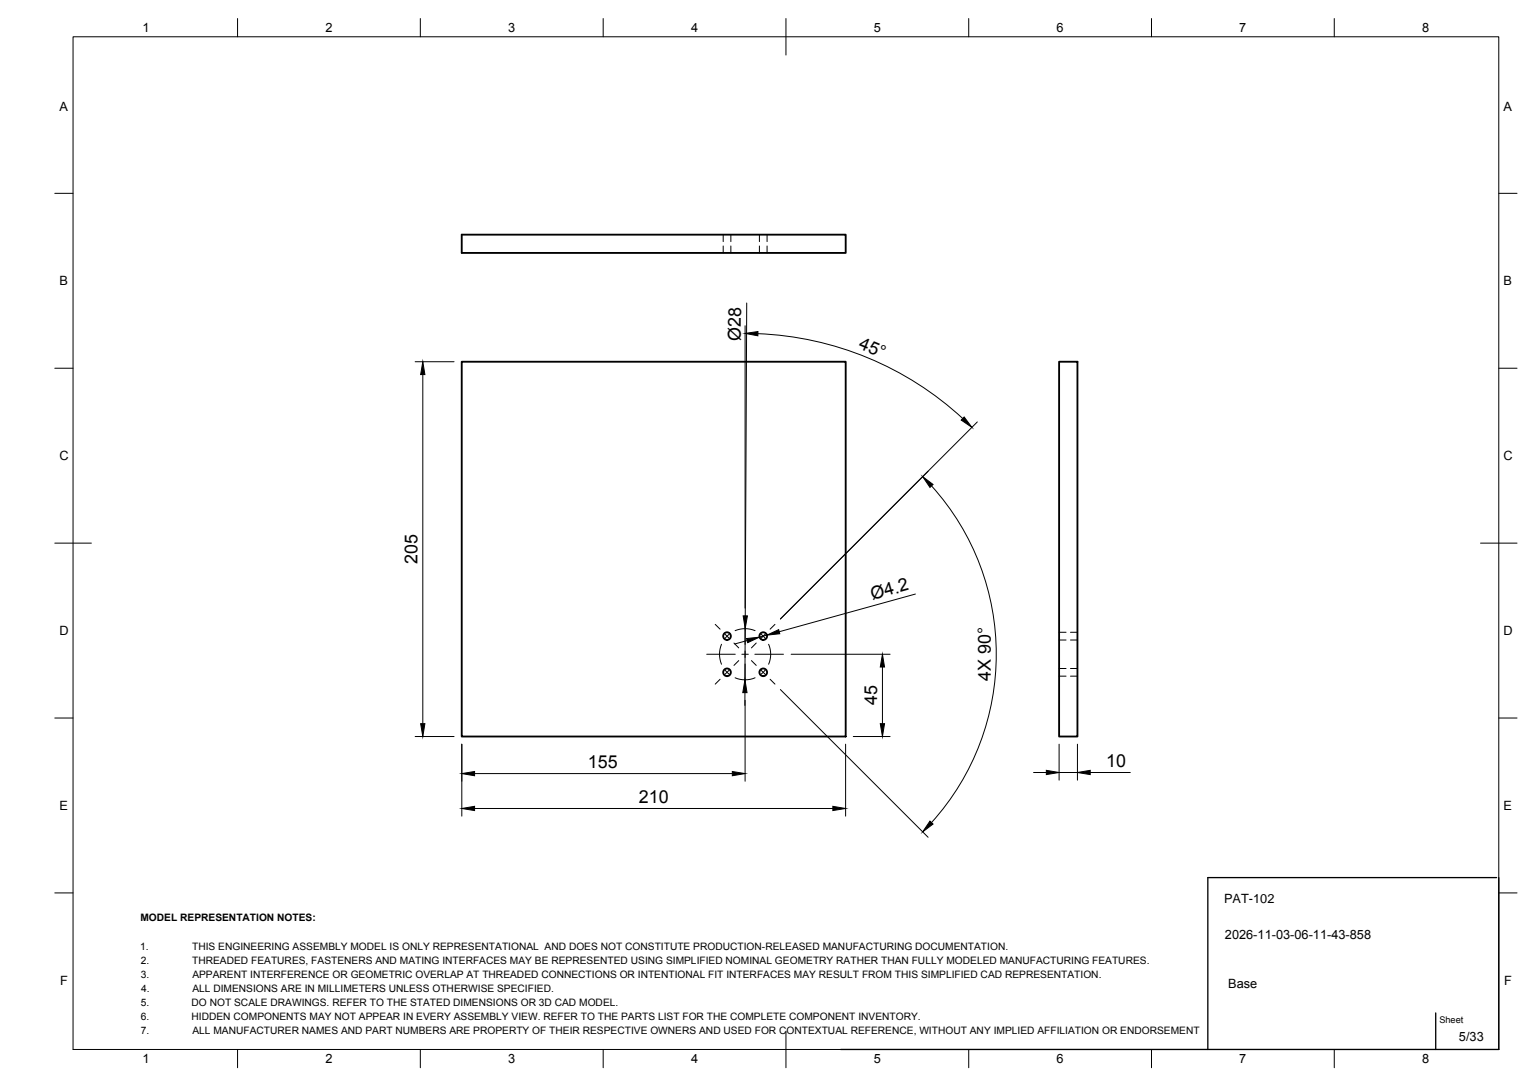
ISO-10303-21;
HEADER;
/* Generated by software containing ST-Developer
 * from STEP Tools, Inc. (www.steptools.com) 
 */

FILE_DESCRIPTION(
/* description */ ('Swing-away clamp arm'),
/* implementation_level */ '2;1');

FILE_NAME(
/* name */ 'Base.step',
/* time_stamp */ '2026-10-28T03:26:03-07:00',
/* author */ (''),
/* organization */ (''),
/* preprocessor_version */ 'ST-DEVELOPER v20.2',
/* originating_system */ 'Autodesk Translation Framework v15.17.0.0',
/* authorisation */ '');

FILE_SCHEMA (('AUTOMOTIVE_DESIGN { 1 0 10303 214 3 1 1 }'));
ENDSEC;

DATA;
#10=MECHANICAL_DESIGN_GEOMETRIC_PRESENTATION_REPRESENTATION('',(#293),#10627);
#241=SHAPE_REPRESENTATION_RELATIONSHIP('SRR','None',#10739,#267);
#267=ADVANCED_BREP_SHAPE_REPRESENTATION('',(#327),#10598);
#293=STYLED_ITEM('',(#10944),#327);
#327=MANIFOLD_SOLID_BREP('Body1',#4899);
#358=FACE_BOUND('',#953,.T.);
#359=FACE_BOUND('',#954,.T.);
#360=FACE_BOUND('',#955,.T.);
#361=FACE_BOUND('',#956,.T.);
#362=FACE_BOUND('',#958,.T.);
#363=FACE_BOUND('',#959,.T.);
#364=FACE_BOUND('',#960,.T.);
#365=FACE_BOUND('',#961,.T.);
#458=PLANE('',#5238);
#459=PLANE('',#5239);
#460=PLANE('',#5240);
#461=PLANE('',#5241);
#462=PLANE('',#5242);
#463=PLANE('',#5243);
#637=FACE_OUTER_BOUND('',#944,.T.);
#638=FACE_OUTER_BOUND('',#945,.T.);
#639=FACE_OUTER_BOUND('',#946,.T.);
#640=FACE_OUTER_BOUND('',#947,.T.);
#641=FACE_OUTER_BOUND('',#948,.T.);
#642=FACE_OUTER_BOUND('',#949,.T.);
#643=FACE_OUTER_BOUND('',#950,.T.);
#644=FACE_OUTER_BOUND('',#951,.T.);
#645=FACE_OUTER_BOUND('',#952,.T.);
#646=FACE_OUTER_BOUND('',#957,.T.);
#944=EDGE_LOOP('',(#3281,#3282,#3283,#3284));
#945=EDGE_LOOP('',(#3285,#3286,#3287,#3288));
#946=EDGE_LOOP('',(#3289,#3290,#3291,#3292));
#947=EDGE_LOOP('',(#3293,#3294,#3295,#3296));
#948=EDGE_LOOP('',(#3297,#3298,#3299,#3300));
#949=EDGE_LOOP('',(#3301,#3302,#3303,#3304));
#950=EDGE_LOOP('',(#3305,#3306,#3307,#3308));
#951=EDGE_LOOP('',(#3309,#3310,#3311,#3312));
#952=EDGE_LOOP('',(#3313,#3314,#3315,#3316));
#953=EDGE_LOOP('',(#3317));
#954=EDGE_LOOP('',(#3318));
#955=EDGE_LOOP('',(#3319));
#956=EDGE_LOOP('',(#3320));
#957=EDGE_LOOP('',(#3321,#3322,#3323,#3324));
#958=EDGE_LOOP('',(#3325));
#959=EDGE_LOOP('',(#3326));
#960=EDGE_LOOP('',(#3327));
#961=EDGE_LOOP('',(#3328));
#1351=LINE('',#7493,#1673);
#1352=LINE('',#7499,#1674);
#1353=LINE('',#7505,#1675);
#1354=LINE('',#7511,#1676);
#1355=LINE('',#7516,#1677);
#1356=LINE('',#7518,#1678);
#1357=LINE('',#7520,#1679);
#1358=LINE('',#7521,#1680);
#1359=LINE('',#7524,#1681);
#1360=LINE('',#7526,#1682);
#1361=LINE('',#7527,#1683);
#1362=LINE('',#7530,#1684);
#1363=LINE('',#7532,#1685);
#1364=LINE('',#7533,#1686);
#1365=LINE('',#7535,#1687);
#1366=LINE('',#7536,#1688);
#1673=VECTOR('',#5880,0.21);
#1674=VECTOR('',#5887,0.21);
#1675=VECTOR('',#5894,0.21);
#1676=VECTOR('',#5901,0.21);
#1677=VECTOR('',#5906,1.);
#1678=VECTOR('',#5907,1.);
#1679=VECTOR('',#5908,1.);
#1680=VECTOR('',#5909,1.);
#1681=VECTOR('',#5912,1.);
#1682=VECTOR('',#5913,1.);
#1683=VECTOR('',#5914,1.);
#1684=VECTOR('',#5917,1.);
#1685=VECTOR('',#5918,1.);
#1686=VECTOR('',#5919,1.);
#1687=VECTOR('',#5922,1.);
#1688=VECTOR('',#5923,1.);
#1995=CIRCLE('',#5227,0.21);
#1996=CIRCLE('',#5228,0.21);
#1997=CIRCLE('',#5230,0.21);
#1998=CIRCLE('',#5231,0.21);
#1999=CIRCLE('',#5233,0.21);
#2000=CIRCLE('',#5234,0.21);
#2001=CIRCLE('',#5236,0.21);
#2002=CIRCLE('',#5237,0.21);
#2262=VERTEX_POINT('',#7490);
#2263=VERTEX_POINT('',#7492);
#2264=VERTEX_POINT('',#7496);
#2265=VERTEX_POINT('',#7498);
#2266=VERTEX_POINT('',#7502);
#2267=VERTEX_POINT('',#7504);
#2268=VERTEX_POINT('',#7508);
#2269=VERTEX_POINT('',#7510);
#2270=VERTEX_POINT('',#7514);
#2271=VERTEX_POINT('',#7515);
#2272=VERTEX_POINT('',#7517);
#2273=VERTEX_POINT('',#7519);
#2274=VERTEX_POINT('',#7523);
#2275=VERTEX_POINT('',#7525);
#2276=VERTEX_POINT('',#7529);
#2277=VERTEX_POINT('',#7531);
#2673=EDGE_CURVE('',#2262,#2262,#1995,.T.);
#2674=EDGE_CURVE('',#2262,#2263,#1351,.T.);
#2675=EDGE_CURVE('',#2263,#2263,#1996,.T.);
#2676=EDGE_CURVE('',#2264,#2264,#1997,.T.);
#2677=EDGE_CURVE('',#2264,#2265,#1352,.T.);
#2678=EDGE_CURVE('',#2265,#2265,#1998,.T.);
#2679=EDGE_CURVE('',#2266,#2266,#1999,.T.);
#2680=EDGE_CURVE('',#2266,#2267,#1353,.T.);
#2681=EDGE_CURVE('',#2267,#2267,#2000,.T.);
#2682=EDGE_CURVE('',#2268,#2268,#2001,.T.);
#2683=EDGE_CURVE('',#2268,#2269,#1354,.T.);
#2684=EDGE_CURVE('',#2269,#2269,#2002,.T.);
#2685=EDGE_CURVE('',#2270,#2271,#1355,.T.);
#2686=EDGE_CURVE('',#2271,#2272,#1356,.T.);
#2687=EDGE_CURVE('',#2273,#2272,#1357,.T.);
#2688=EDGE_CURVE('',#2270,#2273,#1358,.T.);
#2689=EDGE_CURVE('',#2274,#2270,#1359,.T.);
#2690=EDGE_CURVE('',#2275,#2273,#1360,.T.);
#2691=EDGE_CURVE('',#2274,#2275,#1361,.T.);
#2692=EDGE_CURVE('',#2276,#2274,#1362,.T.);
#2693=EDGE_CURVE('',#2277,#2275,#1363,.T.);
#2694=EDGE_CURVE('',#2276,#2277,#1364,.T.);
#2695=EDGE_CURVE('',#2271,#2276,#1365,.T.);
#2696=EDGE_CURVE('',#2272,#2277,#1366,.T.);
#3281=ORIENTED_EDGE('',*,*,#2673,.F.);
#3282=ORIENTED_EDGE('',*,*,#2674,.T.);
#3283=ORIENTED_EDGE('',*,*,#2675,.F.);
#3284=ORIENTED_EDGE('',*,*,#2674,.F.);
#3285=ORIENTED_EDGE('',*,*,#2676,.F.);
#3286=ORIENTED_EDGE('',*,*,#2677,.T.);
#3287=ORIENTED_EDGE('',*,*,#2678,.F.);
#3288=ORIENTED_EDGE('',*,*,#2677,.F.);
#3289=ORIENTED_EDGE('',*,*,#2679,.F.);
#3290=ORIENTED_EDGE('',*,*,#2680,.T.);
#3291=ORIENTED_EDGE('',*,*,#2681,.F.);
#3292=ORIENTED_EDGE('',*,*,#2680,.F.);
#3293=ORIENTED_EDGE('',*,*,#2682,.F.);
#3294=ORIENTED_EDGE('',*,*,#2683,.T.);
#3295=ORIENTED_EDGE('',*,*,#2684,.F.);
#3296=ORIENTED_EDGE('',*,*,#2683,.F.);
#3297=ORIENTED_EDGE('',*,*,#2685,.T.);
#3298=ORIENTED_EDGE('',*,*,#2686,.T.);
#3299=ORIENTED_EDGE('',*,*,#2687,.F.);
#3300=ORIENTED_EDGE('',*,*,#2688,.F.);
#3301=ORIENTED_EDGE('',*,*,#2689,.T.);
#3302=ORIENTED_EDGE('',*,*,#2688,.T.);
#3303=ORIENTED_EDGE('',*,*,#2690,.F.);
#3304=ORIENTED_EDGE('',*,*,#2691,.F.);
#3305=ORIENTED_EDGE('',*,*,#2692,.T.);
#3306=ORIENTED_EDGE('',*,*,#2691,.T.);
#3307=ORIENTED_EDGE('',*,*,#2693,.F.);
#3308=ORIENTED_EDGE('',*,*,#2694,.F.);
#3309=ORIENTED_EDGE('',*,*,#2695,.T.);
#3310=ORIENTED_EDGE('',*,*,#2694,.T.);
#3311=ORIENTED_EDGE('',*,*,#2696,.F.);
#3312=ORIENTED_EDGE('',*,*,#2686,.F.);
#3313=ORIENTED_EDGE('',*,*,#2696,.T.);
#3314=ORIENTED_EDGE('',*,*,#2693,.T.);
#3315=ORIENTED_EDGE('',*,*,#2690,.T.);
#3316=ORIENTED_EDGE('',*,*,#2687,.T.);
#3317=ORIENTED_EDGE('',*,*,#2675,.T.);
#3318=ORIENTED_EDGE('',*,*,#2678,.T.);
#3319=ORIENTED_EDGE('',*,*,#2681,.T.);
#3320=ORIENTED_EDGE('',*,*,#2684,.T.);
#3321=ORIENTED_EDGE('',*,*,#2695,.F.);
#3322=ORIENTED_EDGE('',*,*,#2685,.F.);
#3323=ORIENTED_EDGE('',*,*,#2689,.F.);
#3324=ORIENTED_EDGE('',*,*,#2692,.F.);
#3325=ORIENTED_EDGE('',*,*,#2673,.T.);
#3326=ORIENTED_EDGE('',*,*,#2676,.T.);
#3327=ORIENTED_EDGE('',*,*,#2679,.T.);
#3328=ORIENTED_EDGE('',*,*,#2682,.T.);
#4497=CYLINDRICAL_SURFACE('',#5226,0.21);
#4498=CYLINDRICAL_SURFACE('',#5229,0.21);
#4499=CYLINDRICAL_SURFACE('',#5232,0.21);
#4500=CYLINDRICAL_SURFACE('',#5235,0.21);
#4592=ADVANCED_FACE('',(#637),#4497,.F.);
#4593=ADVANCED_FACE('',(#638),#4498,.F.);
#4594=ADVANCED_FACE('',(#639),#4499,.F.);
#4595=ADVANCED_FACE('',(#640),#4500,.F.);
#4596=ADVANCED_FACE('',(#641),#458,.T.);
#4597=ADVANCED_FACE('',(#642),#459,.T.);
#4598=ADVANCED_FACE('',(#643),#460,.T.);
#4599=ADVANCED_FACE('',(#644),#461,.T.);
#4600=ADVANCED_FACE('',(#645,#358,#359,#360,#361),#462,.T.);
#4601=ADVANCED_FACE('',(#646,#362,#363,#364,#365),#463,.F.);
#4899=CLOSED_SHELL('',(#4592,#4593,#4594,#4595,#4596,#4597,#4598,#4599,
#4600,#4601));
#5225=AXIS2_PLACEMENT_3D('',#7488,#5874,#5875);
#5226=AXIS2_PLACEMENT_3D('',#7489,#5876,#5877);
#5227=AXIS2_PLACEMENT_3D('',#7491,#5878,#5879);
#5228=AXIS2_PLACEMENT_3D('',#7494,#5881,#5882);
#5229=AXIS2_PLACEMENT_3D('',#7495,#5883,#5884);
#5230=AXIS2_PLACEMENT_3D('',#7497,#5885,#5886);
#5231=AXIS2_PLACEMENT_3D('',#7500,#5888,#5889);
#5232=AXIS2_PLACEMENT_3D('',#7501,#5890,#5891);
#5233=AXIS2_PLACEMENT_3D('',#7503,#5892,#5893);
#5234=AXIS2_PLACEMENT_3D('',#7506,#5895,#5896);
#5235=AXIS2_PLACEMENT_3D('',#7507,#5897,#5898);
#5236=AXIS2_PLACEMENT_3D('',#7509,#5899,#5900);
#5237=AXIS2_PLACEMENT_3D('',#7512,#5902,#5903);
#5238=AXIS2_PLACEMENT_3D('',#7513,#5904,#5905);
#5239=AXIS2_PLACEMENT_3D('',#7522,#5910,#5911);
#5240=AXIS2_PLACEMENT_3D('',#7528,#5915,#5916);
#5241=AXIS2_PLACEMENT_3D('',#7534,#5920,#5921);
#5242=AXIS2_PLACEMENT_3D('',#7537,#5924,#5925);
#5243=AXIS2_PLACEMENT_3D('',#7538,#5926,#5927);
#5874=DIRECTION('axis',(0.,0.,1.));
#5875=DIRECTION('refdir',(1.,0.,0.));
#5876=DIRECTION('center_axis',(0.,0.,1.));
#5877=DIRECTION('ref_axis',(1.,0.,0.));
#5878=DIRECTION('center_axis',(0.,0.,1.));
#5879=DIRECTION('ref_axis',(1.,0.,0.));
#5880=DIRECTION('',(0.,0.,1.));
#5881=DIRECTION('center_axis',(0.,0.,-1.));
#5882=DIRECTION('ref_axis',(1.,0.,0.));
#5883=DIRECTION('center_axis',(0.,0.,1.));
#5884=DIRECTION('ref_axis',(1.,0.,0.));
#5885=DIRECTION('center_axis',(0.,0.,1.));
#5886=DIRECTION('ref_axis',(1.,0.,0.));
#5887=DIRECTION('',(0.,0.,1.));
#5888=DIRECTION('center_axis',(0.,0.,-1.));
#5889=DIRECTION('ref_axis',(1.,0.,0.));
#5890=DIRECTION('center_axis',(0.,0.,1.));
#5891=DIRECTION('ref_axis',(1.,0.,0.));
#5892=DIRECTION('center_axis',(0.,0.,1.));
#5893=DIRECTION('ref_axis',(1.,0.,0.));
#5894=DIRECTION('',(0.,0.,1.));
#5895=DIRECTION('center_axis',(0.,0.,-1.));
#5896=DIRECTION('ref_axis',(1.,0.,0.));
#5897=DIRECTION('center_axis',(0.,0.,1.));
#5898=DIRECTION('ref_axis',(1.,0.,0.));
#5899=DIRECTION('center_axis',(0.,0.,1.));
#5900=DIRECTION('ref_axis',(1.,0.,0.));
#5901=DIRECTION('',(0.,0.,1.));
#5902=DIRECTION('center_axis',(0.,0.,-1.));
#5903=DIRECTION('ref_axis',(1.,0.,0.));
#5904=DIRECTION('center_axis',(0.,1.,0.));
#5905=DIRECTION('ref_axis',(-1.,0.,0.));
#5906=DIRECTION('',(-1.,0.,0.));
#5907=DIRECTION('',(0.,0.,1.));
#5908=DIRECTION('',(-1.,0.,0.));
#5909=DIRECTION('',(0.,0.,1.));
#5910=DIRECTION('center_axis',(1.,0.,0.));
#5911=DIRECTION('ref_axis',(0.,1.,0.));
#5912=DIRECTION('',(0.,1.,0.));
#5913=DIRECTION('',(0.,1.,0.));
#5914=DIRECTION('',(0.,0.,1.));
#5915=DIRECTION('center_axis',(0.,-1.,0.));
#5916=DIRECTION('ref_axis',(1.,0.,0.));
#5917=DIRECTION('',(1.,0.,0.));
#5918=DIRECTION('',(1.,0.,0.));
#5919=DIRECTION('',(0.,0.,1.));
#5920=DIRECTION('center_axis',(-1.,0.,0.));
#5921=DIRECTION('ref_axis',(0.,-1.,0.));
#5922=DIRECTION('',(0.,-1.,0.));
#5923=DIRECTION('',(0.,-1.,0.));
#5924=DIRECTION('center_axis',(0.,0.,1.));
#5925=DIRECTION('ref_axis',(1.,0.,0.));
#5926=DIRECTION('center_axis',(0.,0.,1.));
#5927=DIRECTION('ref_axis',(1.,0.,0.));
#7488=CARTESIAN_POINT('',(0.,0.,0.));
#7489=CARTESIAN_POINT('Origin',(-0.989949493661167,-0.989949493661166,-0.1));
#7490=CARTESIAN_POINT('',(-1.19994949366117,-0.989949493661166,0.));
#7491=CARTESIAN_POINT('Origin',(-0.989949493661167,-0.989949493661166,0.));
#7492=CARTESIAN_POINT('',(-1.19994949366117,-0.989949493661166,1.));
#7493=CARTESIAN_POINT('',(-1.19994949366117,-0.989949493661166,-0.1));
#7494=CARTESIAN_POINT('Origin',(-0.989949493661167,-0.989949493661166,1.));
#7495=CARTESIAN_POINT('Origin',(-0.989949493661166,0.989949493661167,-0.1));
#7496=CARTESIAN_POINT('',(-1.19994949366117,0.989949493661167,0.));
#7497=CARTESIAN_POINT('Origin',(-0.989949493661166,0.989949493661167,0.));
#7498=CARTESIAN_POINT('',(-1.19994949366117,0.989949493661167,1.));
#7499=CARTESIAN_POINT('',(-1.19994949366117,0.989949493661167,-0.1));
#7500=CARTESIAN_POINT('Origin',(-0.989949493661166,0.989949493661167,1.));
#7501=CARTESIAN_POINT('Origin',(0.989949493661167,0.989949493661166,-0.1));
#7502=CARTESIAN_POINT('',(0.779949493661167,0.989949493661166,0.));
#7503=CARTESIAN_POINT('Origin',(0.989949493661167,0.989949493661166,0.));
#7504=CARTESIAN_POINT('',(0.779949493661167,0.989949493661166,1.));
#7505=CARTESIAN_POINT('',(0.779949493661167,0.989949493661166,-0.1));
#7506=CARTESIAN_POINT('Origin',(0.989949493661167,0.989949493661166,1.));
#7507=CARTESIAN_POINT('Origin',(0.989949493661166,-0.989949493661167,-0.1));
#7508=CARTESIAN_POINT('',(0.779949493661166,-0.989949493661167,0.));
#7509=CARTESIAN_POINT('Origin',(0.989949493661166,-0.989949493661167,0.));
#7510=CARTESIAN_POINT('',(0.779949493661166,-0.989949493661167,1.));
#7511=CARTESIAN_POINT('',(0.779949493661166,-0.989949493661167,-0.1));
#7512=CARTESIAN_POINT('Origin',(0.989949493661166,-0.989949493661167,1.));
#7513=CARTESIAN_POINT('Origin',(16.,15.5,0.));
#7514=CARTESIAN_POINT('',(16.,15.5,0.));
#7515=CARTESIAN_POINT('',(-4.5,15.5,0.));
#7516=CARTESIAN_POINT('',(16.,15.5,0.));
#7517=CARTESIAN_POINT('',(-4.5,15.5,1.));
#7518=CARTESIAN_POINT('',(-4.5,15.5,0.));
#7519=CARTESIAN_POINT('',(16.,15.5,1.));
#7520=CARTESIAN_POINT('',(16.,15.5,1.));
#7521=CARTESIAN_POINT('',(16.,15.5,0.));
#7522=CARTESIAN_POINT('Origin',(16.,-5.5,0.));
#7523=CARTESIAN_POINT('',(16.,-5.5,0.));
#7524=CARTESIAN_POINT('',(16.,-5.5,0.));
#7525=CARTESIAN_POINT('',(16.,-5.5,1.));
#7526=CARTESIAN_POINT('',(16.,-5.5,1.));
#7527=CARTESIAN_POINT('',(16.,-5.5,0.));
#7528=CARTESIAN_POINT('Origin',(-4.5,-5.5,0.));
#7529=CARTESIAN_POINT('',(-4.5,-5.5,0.));
#7530=CARTESIAN_POINT('',(-4.5,-5.5,0.));
#7531=CARTESIAN_POINT('',(-4.5,-5.5,1.));
#7532=CARTESIAN_POINT('',(-4.5,-5.5,1.));
#7533=CARTESIAN_POINT('',(-4.5,-5.5,0.));
#7534=CARTESIAN_POINT('Origin',(-4.5,15.5,0.));
#7535=CARTESIAN_POINT('',(-4.5,15.5,0.));
#7536=CARTESIAN_POINT('',(-4.5,15.5,1.));
#7537=CARTESIAN_POINT('Origin',(5.75,5.,1.));
#7538=CARTESIAN_POINT('Origin',(5.75,5.,0.));
#10566=UNCERTAINTY_MEASURE_WITH_UNIT(LENGTH_MEASURE(0.001),#10628,
'DISTANCE_ACCURACY_VALUE',
'Maximum model space distance between geometric entities at asserted c
onnectivities');
#10595=UNCERTAINTY_MEASURE_WITH_UNIT(LENGTH_MEASURE(0.001),#10628,
'DISTANCE_ACCURACY_VALUE',
'Maximum model space distance between geometric entities at asserted c
onnectivities');
#10598=(
GEOMETRIC_REPRESENTATION_CONTEXT(3)
GLOBAL_UNCERTAINTY_ASSIGNED_CONTEXT((#10566))
GLOBAL_UNIT_ASSIGNED_CONTEXT((#10628,#10630,#10631))
REPRESENTATION_CONTEXT('','3D')
);
#10627=(
GEOMETRIC_REPRESENTATION_CONTEXT(3)
GLOBAL_UNCERTAINTY_ASSIGNED_CONTEXT((#10595))
GLOBAL_UNIT_ASSIGNED_CONTEXT((#10628,#10630,#10631))
REPRESENTATION_CONTEXT('','3D')
);
#10628=(
LENGTH_UNIT()
NAMED_UNIT(*)
SI_UNIT(.CENTI.,.METRE.)
);
#10630=(
NAMED_UNIT(*)
PLANE_ANGLE_UNIT()
SI_UNIT($,.RADIAN.)
);
#10631=(
NAMED_UNIT(*)
SI_UNIT($,.STERADIAN.)
SOLID_ANGLE_UNIT()
);
#10634=SHAPE_DEFINITION_REPRESENTATION(#10665,#10739);
#10665=PRODUCT_DEFINITION_SHAPE('',$,#10771);
#10739=SHAPE_REPRESENTATION('',(#5225),#10598);
#10768=PRODUCT_DEFINITION_CONTEXT('part definition',#10863,'design');
#10771=PRODUCT_DEFINITION('Base','Base',#10802,#10768);
#10802=PRODUCT_DEFINITION_FORMATION('',$,#10867);
#10863=APPLICATION_CONTEXT(
'Core Data for Automotive Mechanical Design Process');
#10864=PRODUCT_CONTEXT('part definition',#10863,'mechanical');
#10867=PRODUCT('Base','Base','Base',(#10864));
#10938=COLOUR_RGB('Dark Blue',0.08,0.2,0.34);
#10939=FILL_AREA_STYLE_COLOUR('',#10938);
#10940=FILL_AREA_STYLE('',(#10939));
#10941=SURFACE_STYLE_FILL_AREA(#10940);
#10942=SURFACE_SIDE_STYLE('',(#10941));
#10943=SURFACE_STYLE_USAGE(.BOTH.,#10942);
#10944=PRESENTATION_STYLE_ASSIGNMENT((#10943));
ENDSEC;
END-ISO-10303-21;
